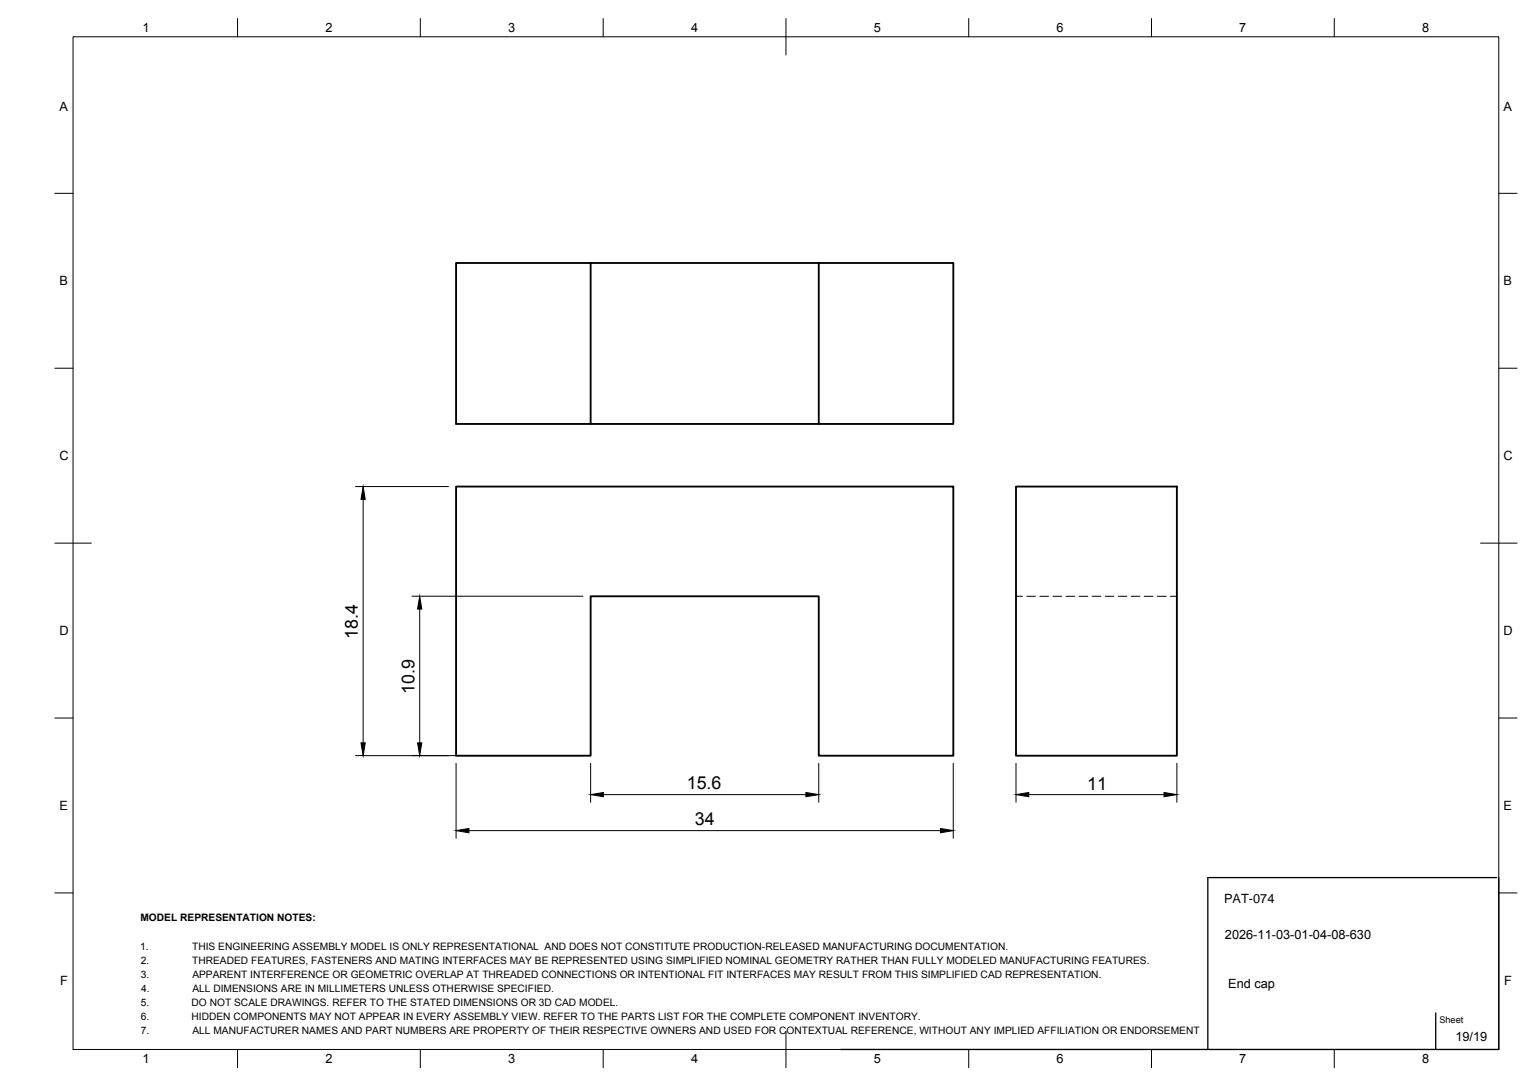
ISO-10303-21;
HEADER;
/* Generated by software containing ST-Developer
 * from STEP Tools, Inc. (www.steptools.com) 
 */

FILE_DESCRIPTION(
/* description */ ('Manual rail carriage with stops'),
/* implementation_level */ '2;1');

FILE_NAME(
/* name */ 'End cap.step',
/* time_stamp */ '2026-10-27T18:54:27-07:00',
/* author */ (''),
/* organization */ (''),
/* preprocessor_version */ 'ST-DEVELOPER v20.2',
/* originating_system */ 'Autodesk Translation Framework v15.17.0.0',
/* authorisation */ '');

FILE_SCHEMA (('AUTOMOTIVE_DESIGN { 1 0 10303 214 3 1 1 }'));
ENDSEC;

DATA;
#10=MECHANICAL_DESIGN_GEOMETRIC_PRESENTATION_REPRESENTATION('',(#284),#8499);
#248=SHAPE_REPRESENTATION_RELATIONSHIP('SRR','None',#8613,#266);
#266=ADVANCED_BREP_SHAPE_REPRESENTATION('',(#300),#8492);
#284=STYLED_ITEM('',(#8802),#300);
#300=MANIFOLD_SOLID_BREP('Body1',#4954);
#533=PLANE('',#5465);
#534=PLANE('',#5466);
#535=PLANE('',#5467);
#536=PLANE('',#5468);
#537=PLANE('',#5469);
#538=PLANE('',#5470);
#539=PLANE('',#5471);
#540=PLANE('',#5472);
#541=PLANE('',#5473);
#542=PLANE('',#5474);
#773=FACE_OUTER_BOUND('',#1093,.T.);
#774=FACE_OUTER_BOUND('',#1094,.T.);
#775=FACE_OUTER_BOUND('',#1095,.T.);
#776=FACE_OUTER_BOUND('',#1096,.T.);
#777=FACE_OUTER_BOUND('',#1097,.T.);
#778=FACE_OUTER_BOUND('',#1098,.T.);
#779=FACE_OUTER_BOUND('',#1099,.T.);
#780=FACE_OUTER_BOUND('',#1100,.T.);
#781=FACE_OUTER_BOUND('',#1101,.T.);
#782=FACE_OUTER_BOUND('',#1102,.T.);
#1093=EDGE_LOOP('',(#4348,#4349,#4350,#4351));
#1094=EDGE_LOOP('',(#4352,#4353,#4354,#4355));
#1095=EDGE_LOOP('',(#4356,#4357,#4358,#4359));
#1096=EDGE_LOOP('',(#4360,#4361,#4362,#4363));
#1097=EDGE_LOOP('',(#4364,#4365,#4366,#4367));
#1098=EDGE_LOOP('',(#4368,#4369,#4370,#4371));
#1099=EDGE_LOOP('',(#4372,#4373,#4374,#4375));
#1100=EDGE_LOOP('',(#4376,#4377,#4378,#4379));
#1101=EDGE_LOOP('',(#4380,#4381,#4382,#4383,#4384,#4385,#4386,#4387));
#1102=EDGE_LOOP('',(#4388,#4389,#4390,#4391,#4392,#4393,#4394,#4395));
#1585=LINE('',#8105,#2085);
#1586=LINE('',#8107,#2086);
#1587=LINE('',#8109,#2087);
#1588=LINE('',#8110,#2088);
#1589=LINE('',#8113,#2089);
#1590=LINE('',#8115,#2090);
#1591=LINE('',#8116,#2091);
#1592=LINE('',#8119,#2092);
#1593=LINE('',#8121,#2093);
#1594=LINE('',#8122,#2094);
#1595=LINE('',#8125,#2095);
#1596=LINE('',#8127,#2096);
#1597=LINE('',#8128,#2097);
#1598=LINE('',#8131,#2098);
#1599=LINE('',#8133,#2099);
#1600=LINE('',#8134,#2100);
#1601=LINE('',#8137,#2101);
#1602=LINE('',#8139,#2102);
#1603=LINE('',#8140,#2103);
#1604=LINE('',#8143,#2104);
#1605=LINE('',#8145,#2105);
#1606=LINE('',#8146,#2106);
#1607=LINE('',#8148,#2107);
#1608=LINE('',#8149,#2108);
#2085=VECTOR('',#6642,1.);
#2086=VECTOR('',#6643,1.);
#2087=VECTOR('',#6644,1.);
#2088=VECTOR('',#6645,1.);
#2089=VECTOR('',#6648,1.);
#2090=VECTOR('',#6649,1.);
#2091=VECTOR('',#6650,1.);
#2092=VECTOR('',#6653,1.);
#2093=VECTOR('',#6654,1.);
#2094=VECTOR('',#6655,1.);
#2095=VECTOR('',#6658,1.);
#2096=VECTOR('',#6659,1.);
#2097=VECTOR('',#6660,1.);
#2098=VECTOR('',#6663,1.);
#2099=VECTOR('',#6664,1.);
#2100=VECTOR('',#6665,1.);
#2101=VECTOR('',#6668,1.);
#2102=VECTOR('',#6669,1.);
#2103=VECTOR('',#6670,1.);
#2104=VECTOR('',#6673,1.);
#2105=VECTOR('',#6674,1.);
#2106=VECTOR('',#6675,1.);
#2107=VECTOR('',#6678,1.);
#2108=VECTOR('',#6679,1.);
#2639=VERTEX_POINT('',#8103);
#2640=VERTEX_POINT('',#8104);
#2641=VERTEX_POINT('',#8106);
#2642=VERTEX_POINT('',#8108);
#2643=VERTEX_POINT('',#8112);
#2644=VERTEX_POINT('',#8114);
#2645=VERTEX_POINT('',#8118);
#2646=VERTEX_POINT('',#8120);
#2647=VERTEX_POINT('',#8124);
#2648=VERTEX_POINT('',#8126);
#2649=VERTEX_POINT('',#8130);
#2650=VERTEX_POINT('',#8132);
#2651=VERTEX_POINT('',#8136);
#2652=VERTEX_POINT('',#8138);
#2653=VERTEX_POINT('',#8142);
#2654=VERTEX_POINT('',#8144);
#3222=EDGE_CURVE('',#2639,#2640,#1585,.T.);
#3223=EDGE_CURVE('',#2639,#2641,#1586,.T.);
#3224=EDGE_CURVE('',#2642,#2641,#1587,.T.);
#3225=EDGE_CURVE('',#2640,#2642,#1588,.T.);
#3226=EDGE_CURVE('',#2640,#2643,#1589,.T.);
#3227=EDGE_CURVE('',#2644,#2642,#1590,.T.);
#3228=EDGE_CURVE('',#2643,#2644,#1591,.T.);
#3229=EDGE_CURVE('',#2643,#2645,#1592,.T.);
#3230=EDGE_CURVE('',#2646,#2644,#1593,.T.);
#3231=EDGE_CURVE('',#2645,#2646,#1594,.T.);
#3232=EDGE_CURVE('',#2645,#2647,#1595,.T.);
#3233=EDGE_CURVE('',#2648,#2646,#1596,.T.);
#3234=EDGE_CURVE('',#2647,#2648,#1597,.T.);
#3235=EDGE_CURVE('',#2647,#2649,#1598,.T.);
#3236=EDGE_CURVE('',#2650,#2648,#1599,.T.);
#3237=EDGE_CURVE('',#2649,#2650,#1600,.T.);
#3238=EDGE_CURVE('',#2649,#2651,#1601,.T.);
#3239=EDGE_CURVE('',#2652,#2650,#1602,.T.);
#3240=EDGE_CURVE('',#2651,#2652,#1603,.T.);
#3241=EDGE_CURVE('',#2651,#2653,#1604,.T.);
#3242=EDGE_CURVE('',#2654,#2652,#1605,.T.);
#3243=EDGE_CURVE('',#2653,#2654,#1606,.T.);
#3244=EDGE_CURVE('',#2653,#2639,#1607,.T.);
#3245=EDGE_CURVE('',#2641,#2654,#1608,.T.);
#4348=ORIENTED_EDGE('',*,*,#3222,.F.);
#4349=ORIENTED_EDGE('',*,*,#3223,.T.);
#4350=ORIENTED_EDGE('',*,*,#3224,.F.);
#4351=ORIENTED_EDGE('',*,*,#3225,.F.);
#4352=ORIENTED_EDGE('',*,*,#3226,.F.);
#4353=ORIENTED_EDGE('',*,*,#3225,.T.);
#4354=ORIENTED_EDGE('',*,*,#3227,.F.);
#4355=ORIENTED_EDGE('',*,*,#3228,.F.);
#4356=ORIENTED_EDGE('',*,*,#3229,.F.);
#4357=ORIENTED_EDGE('',*,*,#3228,.T.);
#4358=ORIENTED_EDGE('',*,*,#3230,.F.);
#4359=ORIENTED_EDGE('',*,*,#3231,.F.);
#4360=ORIENTED_EDGE('',*,*,#3232,.F.);
#4361=ORIENTED_EDGE('',*,*,#3231,.T.);
#4362=ORIENTED_EDGE('',*,*,#3233,.F.);
#4363=ORIENTED_EDGE('',*,*,#3234,.F.);
#4364=ORIENTED_EDGE('',*,*,#3235,.F.);
#4365=ORIENTED_EDGE('',*,*,#3234,.T.);
#4366=ORIENTED_EDGE('',*,*,#3236,.F.);
#4367=ORIENTED_EDGE('',*,*,#3237,.F.);
#4368=ORIENTED_EDGE('',*,*,#3238,.F.);
#4369=ORIENTED_EDGE('',*,*,#3237,.T.);
#4370=ORIENTED_EDGE('',*,*,#3239,.F.);
#4371=ORIENTED_EDGE('',*,*,#3240,.F.);
#4372=ORIENTED_EDGE('',*,*,#3241,.F.);
#4373=ORIENTED_EDGE('',*,*,#3240,.T.);
#4374=ORIENTED_EDGE('',*,*,#3242,.F.);
#4375=ORIENTED_EDGE('',*,*,#3243,.F.);
#4376=ORIENTED_EDGE('',*,*,#3244,.F.);
#4377=ORIENTED_EDGE('',*,*,#3243,.T.);
#4378=ORIENTED_EDGE('',*,*,#3245,.F.);
#4379=ORIENTED_EDGE('',*,*,#3223,.F.);
#4380=ORIENTED_EDGE('',*,*,#3244,.T.);
#4381=ORIENTED_EDGE('',*,*,#3222,.T.);
#4382=ORIENTED_EDGE('',*,*,#3226,.T.);
#4383=ORIENTED_EDGE('',*,*,#3229,.T.);
#4384=ORIENTED_EDGE('',*,*,#3232,.T.);
#4385=ORIENTED_EDGE('',*,*,#3235,.T.);
#4386=ORIENTED_EDGE('',*,*,#3238,.T.);
#4387=ORIENTED_EDGE('',*,*,#3241,.T.);
#4388=ORIENTED_EDGE('',*,*,#3245,.T.);
#4389=ORIENTED_EDGE('',*,*,#3242,.T.);
#4390=ORIENTED_EDGE('',*,*,#3239,.T.);
#4391=ORIENTED_EDGE('',*,*,#3236,.T.);
#4392=ORIENTED_EDGE('',*,*,#3233,.T.);
#4393=ORIENTED_EDGE('',*,*,#3230,.T.);
#4394=ORIENTED_EDGE('',*,*,#3227,.T.);
#4395=ORIENTED_EDGE('',*,*,#3224,.T.);
#4872=ADVANCED_FACE('',(#773),#533,.T.);
#4873=ADVANCED_FACE('',(#774),#534,.T.);
#4874=ADVANCED_FACE('',(#775),#535,.T.);
#4875=ADVANCED_FACE('',(#776),#536,.T.);
#4876=ADVANCED_FACE('',(#777),#537,.T.);
#4877=ADVANCED_FACE('',(#778),#538,.T.);
#4878=ADVANCED_FACE('',(#779),#539,.T.);
#4879=ADVANCED_FACE('',(#780),#540,.T.);
#4880=ADVANCED_FACE('',(#781),#541,.T.);
#4881=ADVANCED_FACE('',(#782),#542,.T.);
#4954=CLOSED_SHELL('',(#4872,#4873,#4874,#4875,#4876,#4877,#4878,#4879,
#4880,#4881));
#5464=AXIS2_PLACEMENT_3D('',#8101,#6638,#6639);
#5465=AXIS2_PLACEMENT_3D('',#8102,#6640,#6641);
#5466=AXIS2_PLACEMENT_3D('',#8111,#6646,#6647);
#5467=AXIS2_PLACEMENT_3D('',#8117,#6651,#6652);
#5468=AXIS2_PLACEMENT_3D('',#8123,#6656,#6657);
#5469=AXIS2_PLACEMENT_3D('',#8129,#6661,#6662);
#5470=AXIS2_PLACEMENT_3D('',#8135,#6666,#6667);
#5471=AXIS2_PLACEMENT_3D('',#8141,#6671,#6672);
#5472=AXIS2_PLACEMENT_3D('',#8147,#6676,#6677);
#5473=AXIS2_PLACEMENT_3D('',#8150,#6680,#6681);
#5474=AXIS2_PLACEMENT_3D('',#8151,#6682,#6683);
#6638=DIRECTION('axis',(0.,0.,1.));
#6639=DIRECTION('refdir',(1.,0.,0.));
#6640=DIRECTION('center_axis',(0.,0.,-1.));
#6641=DIRECTION('ref_axis',(0.,-1.,0.));
#6642=DIRECTION('',(0.,1.,0.));
#6643=DIRECTION('',(-1.,0.,0.));
#6644=DIRECTION('',(0.,-1.,0.));
#6645=DIRECTION('',(-1.,0.,0.));
#6646=DIRECTION('center_axis',(0.,1.,0.));
#6647=DIRECTION('ref_axis',(0.,0.,-1.));
#6648=DIRECTION('',(0.,0.,1.));
#6649=DIRECTION('',(0.,0.,-1.));
#6650=DIRECTION('',(-1.,0.,0.));
#6651=DIRECTION('center_axis',(0.,0.,-1.));
#6652=DIRECTION('ref_axis',(0.,-1.,0.));
#6653=DIRECTION('',(0.,1.,0.));
#6654=DIRECTION('',(0.,-1.,0.));
#6655=DIRECTION('',(-1.,0.,0.));
#6656=DIRECTION('center_axis',(0.,-1.,0.));
#6657=DIRECTION('ref_axis',(0.,0.,1.));
#6658=DIRECTION('',(0.,0.,-1.));
#6659=DIRECTION('',(0.,0.,1.));
#6660=DIRECTION('',(-1.,0.,0.));
#6661=DIRECTION('center_axis',(0.,0.,-1.));
#6662=DIRECTION('ref_axis',(0.,-1.,0.));
#6663=DIRECTION('',(0.,1.,0.));
#6664=DIRECTION('',(0.,-1.,0.));
#6665=DIRECTION('',(-1.,0.,0.));
#6666=DIRECTION('center_axis',(0.,1.,0.));
#6667=DIRECTION('ref_axis',(0.,0.,-1.));
#6668=DIRECTION('',(0.,0.,1.));
#6669=DIRECTION('',(0.,0.,-1.));
#6670=DIRECTION('',(-1.,0.,0.));
#6671=DIRECTION('center_axis',(0.,0.,1.));
#6672=DIRECTION('ref_axis',(0.,1.,0.));
#6673=DIRECTION('',(0.,-1.,0.));
#6674=DIRECTION('',(0.,1.,0.));
#6675=DIRECTION('',(-1.,0.,0.));
#6676=DIRECTION('center_axis',(0.,-1.,0.));
#6677=DIRECTION('ref_axis',(0.,0.,1.));
#6678=DIRECTION('',(0.,0.,-1.));
#6679=DIRECTION('',(0.,0.,1.));
#6680=DIRECTION('center_axis',(1.,0.,0.));
#6681=DIRECTION('ref_axis',(0.,0.,-1.));
#6682=DIRECTION('center_axis',(-1.,0.,0.));
#6683=DIRECTION('ref_axis',(0.,0.,1.));
#8101=CARTESIAN_POINT('',(0.,0.,0.));
#8102=CARTESIAN_POINT('Origin',(-1.97,-0.78,0.46));
#8103=CARTESIAN_POINT('',(-1.97,-1.7,0.46));
#8104=CARTESIAN_POINT('',(-1.97,-0.78,0.46));
#8105=CARTESIAN_POINT('',(-1.97,-1.7,0.46));
#8106=CARTESIAN_POINT('',(-3.07,-1.7,0.46));
#8107=CARTESIAN_POINT('',(-1.97,-1.7,0.46));
#8108=CARTESIAN_POINT('',(-3.07,-0.78,0.46));
#8109=CARTESIAN_POINT('',(-3.07,-1.7,0.46));
#8110=CARTESIAN_POINT('',(-1.97,-0.78,0.46));
#8111=CARTESIAN_POINT('Origin',(-1.97,-0.78,1.55));
#8112=CARTESIAN_POINT('',(-1.97,-0.78,1.55));
#8113=CARTESIAN_POINT('',(-1.97,-0.78,0.46));
#8114=CARTESIAN_POINT('',(-3.07,-0.78,1.55));
#8115=CARTESIAN_POINT('',(-3.07,-0.78,0.46));
#8116=CARTESIAN_POINT('',(-1.97,-0.78,1.55));
#8117=CARTESIAN_POINT('Origin',(-1.97,0.78,1.55));
#8118=CARTESIAN_POINT('',(-1.97,0.78,1.55));
#8119=CARTESIAN_POINT('',(-1.97,-0.78,1.55));
#8120=CARTESIAN_POINT('',(-3.07,0.78,1.55));
#8121=CARTESIAN_POINT('',(-3.07,-0.78,1.55));
#8122=CARTESIAN_POINT('',(-1.97,0.78,1.55));
#8123=CARTESIAN_POINT('Origin',(-1.97,0.78,0.46));
#8124=CARTESIAN_POINT('',(-1.97,0.78,0.46));
#8125=CARTESIAN_POINT('',(-1.97,0.78,1.55));
#8126=CARTESIAN_POINT('',(-3.07,0.78,0.46));
#8127=CARTESIAN_POINT('',(-3.07,0.78,1.55));
#8128=CARTESIAN_POINT('',(-1.97,0.78,0.46));
#8129=CARTESIAN_POINT('Origin',(-1.97,1.7,0.46));
#8130=CARTESIAN_POINT('',(-1.97,1.7,0.46));
#8131=CARTESIAN_POINT('',(-1.97,0.78,0.46));
#8132=CARTESIAN_POINT('',(-3.07,1.7,0.46));
#8133=CARTESIAN_POINT('',(-3.07,0.78,0.46));
#8134=CARTESIAN_POINT('',(-1.97,1.7,0.46));
#8135=CARTESIAN_POINT('Origin',(-1.97,1.7,2.3));
#8136=CARTESIAN_POINT('',(-1.97,1.7,2.3));
#8137=CARTESIAN_POINT('',(-1.97,1.7,0.46));
#8138=CARTESIAN_POINT('',(-3.07,1.7,2.3));
#8139=CARTESIAN_POINT('',(-3.07,1.7,0.46));
#8140=CARTESIAN_POINT('',(-1.97,1.7,2.3));
#8141=CARTESIAN_POINT('Origin',(-1.97,-1.7,2.3));
#8142=CARTESIAN_POINT('',(-1.97,-1.7,2.3));
#8143=CARTESIAN_POINT('',(-1.97,1.7,2.3));
#8144=CARTESIAN_POINT('',(-3.07,-1.7,2.3));
#8145=CARTESIAN_POINT('',(-3.07,1.7,2.3));
#8146=CARTESIAN_POINT('',(-1.97,-1.7,2.3));
#8147=CARTESIAN_POINT('Origin',(-1.97,-1.7,0.46));
#8148=CARTESIAN_POINT('',(-1.97,-1.7,2.3));
#8149=CARTESIAN_POINT('',(-3.07,-1.7,2.3));
#8150=CARTESIAN_POINT('Origin',(-1.97,0.,1.38));
#8151=CARTESIAN_POINT('Origin',(-3.07,0.,1.38));
#8469=UNCERTAINTY_MEASURE_WITH_UNIT(LENGTH_MEASURE(0.001),#8500,
'DISTANCE_ACCURACY_VALUE',
'Maximum model space distance between geometric entities at asserted c
onnectivities');
#8476=UNCERTAINTY_MEASURE_WITH_UNIT(LENGTH_MEASURE(0.001),#8500,
'DISTANCE_ACCURACY_VALUE',
'Maximum model space distance between geometric entities at asserted c
onnectivities');
#8492=(
GEOMETRIC_REPRESENTATION_CONTEXT(3)
GLOBAL_UNCERTAINTY_ASSIGNED_CONTEXT((#8469))
GLOBAL_UNIT_ASSIGNED_CONTEXT((#8500,#8502,#8503))
REPRESENTATION_CONTEXT('','3D')
);
#8499=(
GEOMETRIC_REPRESENTATION_CONTEXT(3)
GLOBAL_UNCERTAINTY_ASSIGNED_CONTEXT((#8476))
GLOBAL_UNIT_ASSIGNED_CONTEXT((#8500,#8502,#8503))
REPRESENTATION_CONTEXT('','3D')
);
#8500=(
LENGTH_UNIT()
NAMED_UNIT(*)
SI_UNIT(.CENTI.,.METRE.)
);
#8502=(
NAMED_UNIT(*)
PLANE_ANGLE_UNIT()
SI_UNIT($,.RADIAN.)
);
#8503=(
NAMED_UNIT(*)
SI_UNIT($,.STERADIAN.)
SOLID_ANGLE_UNIT()
);
#8519=SHAPE_DEFINITION_REPRESENTATION(#8541,#8613);
#8541=PRODUCT_DEFINITION_SHAPE('',$,#8636);
#8613=SHAPE_REPRESENTATION('',(#5464),#8492);
#8620=PRODUCT_DEFINITION_CONTEXT('part definition',#8688,'design');
#8636=PRODUCT_DEFINITION('End cap','End cap',#8658,#8620);
#8658=PRODUCT_DEFINITION_FORMATION('',$,#8705);
#8688=APPLICATION_CONTEXT(
'Core Data for Automotive Mechanical Design Process');
#8689=PRODUCT_CONTEXT('part definition',#8688,'mechanical');
#8705=PRODUCT('End cap','End cap','End cap',(#8689));
#8796=COLOUR_RGB('Off White',0.89,0.88,0.83);
#8797=FILL_AREA_STYLE_COLOUR('',#8796);
#8798=FILL_AREA_STYLE('',(#8797));
#8799=SURFACE_STYLE_FILL_AREA(#8798);
#8800=SURFACE_SIDE_STYLE('',(#8799));
#8801=SURFACE_STYLE_USAGE(.BOTH.,#8800);
#8802=PRESENTATION_STYLE_ASSIGNMENT((#8801));
ENDSEC;
END-ISO-10303-21;
